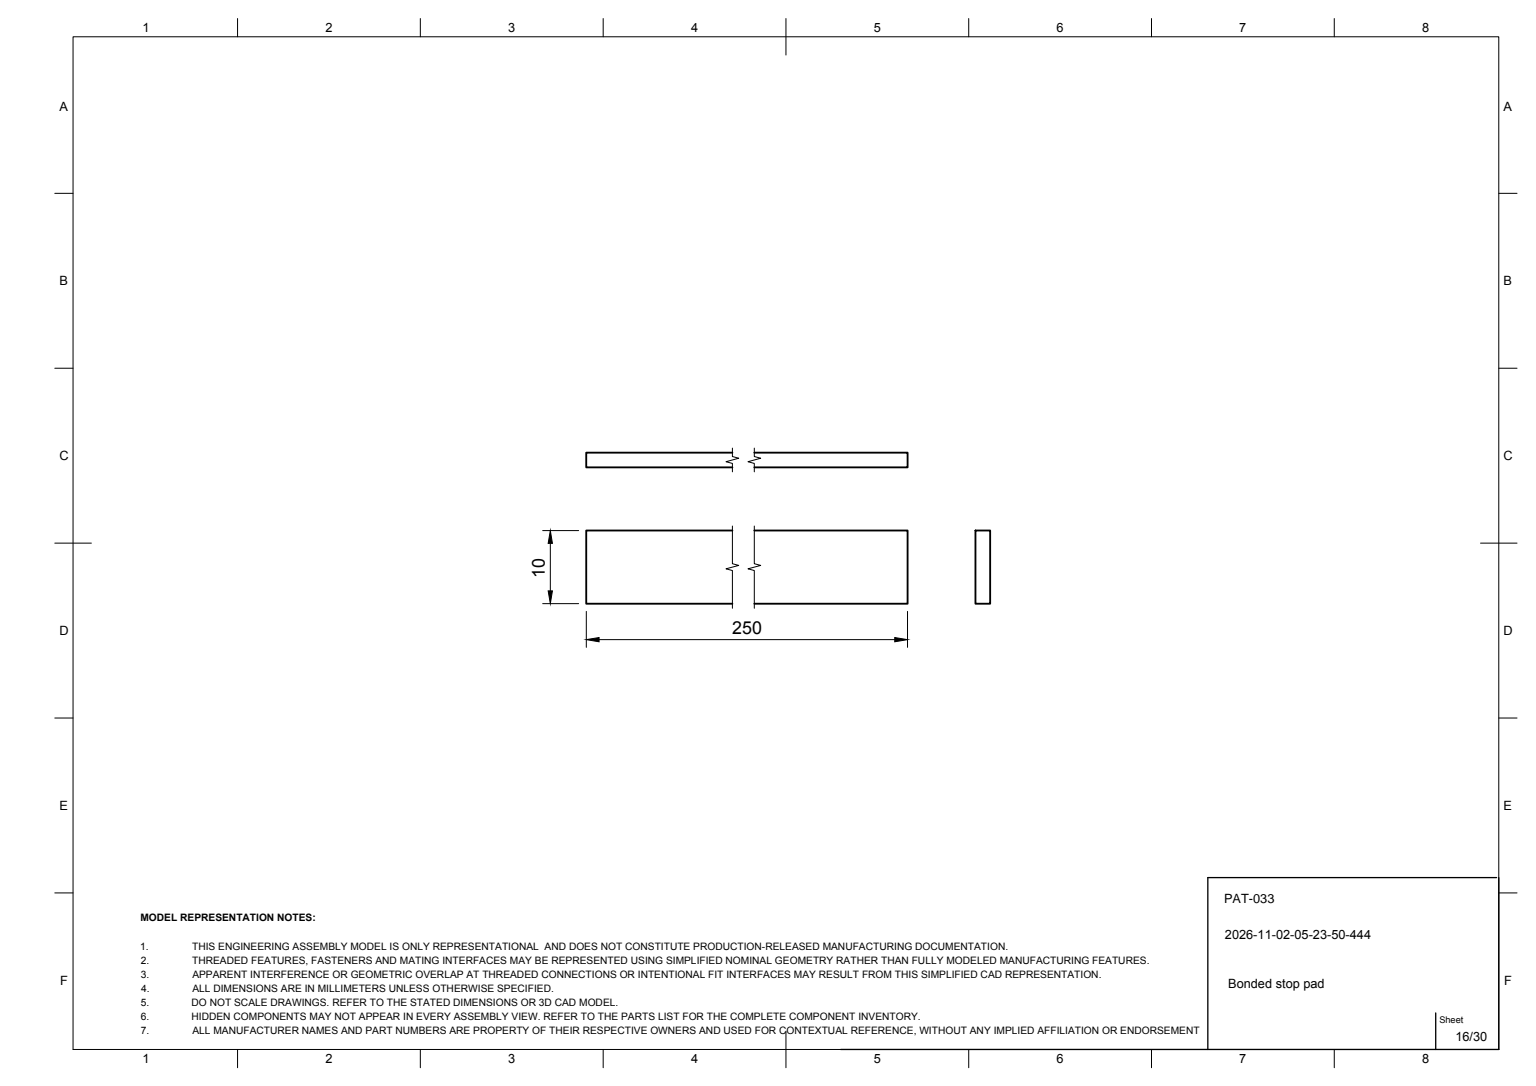
ISO-10303-21;
HEADER;
/* Generated by software containing ST-Developer
 * from STEP Tools, Inc. (www.steptools.com) 
 */

FILE_DESCRIPTION(
/* description */ ('Dual-rail gantry carriage'),
/* implementation_level */ '2;1');

FILE_NAME(
/* name */ 'Bonded stop pad.step',
/* time_stamp */ '2026-10-27T10:49:15-07:00',
/* author */ (''),
/* organization */ (''),
/* preprocessor_version */ 'ST-DEVELOPER v20.2',
/* originating_system */ 'Autodesk Translation Framework v15.17.0.0',
/* authorisation */ '');

FILE_SCHEMA (('AUTOMOTIVE_DESIGN { 1 0 10303 214 3 1 1 }'));
ENDSEC;

DATA;
#10=MECHANICAL_DESIGN_GEOMETRIC_PRESENTATION_REPRESENTATION('',(#596),#12804);
#534=SHAPE_REPRESENTATION_RELATIONSHIP('SRR','None',#13012,#565);
#565=ADVANCED_BREP_SHAPE_REPRESENTATION('',(#627),#12782);
#596=STYLED_ITEM('',(#13261),#627);
#627=MANIFOLD_SOLID_BREP('Body1',#7374);
#834=PLANE('',#7903);
#835=PLANE('',#7904);
#836=PLANE('',#7905);
#837=PLANE('',#7906);
#838=PLANE('',#7907);
#839=PLANE('',#7908);
#1144=FACE_OUTER_BOUND('',#1577,.T.);
#1145=FACE_OUTER_BOUND('',#1578,.T.);
#1146=FACE_OUTER_BOUND('',#1579,.T.);
#1147=FACE_OUTER_BOUND('',#1580,.T.);
#1148=FACE_OUTER_BOUND('',#1581,.T.);
#1149=FACE_OUTER_BOUND('',#1582,.T.);
#1577=EDGE_LOOP('',(#5503,#5504,#5505,#5506));
#1578=EDGE_LOOP('',(#5507,#5508,#5509,#5510));
#1579=EDGE_LOOP('',(#5511,#5512,#5513,#5514));
#1580=EDGE_LOOP('',(#5515,#5516,#5517,#5518));
#1581=EDGE_LOOP('',(#5519,#5520,#5521,#5522));
#1582=EDGE_LOOP('',(#5523,#5524,#5525,#5526));
#2114=LINE('',#11159,#2823);
#2115=LINE('',#11161,#2824);
#2116=LINE('',#11163,#2825);
#2117=LINE('',#11164,#2826);
#2118=LINE('',#11167,#2827);
#2119=LINE('',#11169,#2828);
#2120=LINE('',#11170,#2829);
#2121=LINE('',#11173,#2830);
#2122=LINE('',#11175,#2831);
#2123=LINE('',#11176,#2832);
#2124=LINE('',#11178,#2833);
#2125=LINE('',#11179,#2834);
#2823=VECTOR('',#8979,1.);
#2824=VECTOR('',#8980,1.);
#2825=VECTOR('',#8981,1.);
#2826=VECTOR('',#8982,1.);
#2827=VECTOR('',#8985,1.);
#2828=VECTOR('',#8986,1.);
#2829=VECTOR('',#8987,1.);
#2830=VECTOR('',#8990,1.);
#2831=VECTOR('',#8991,1.);
#2832=VECTOR('',#8992,1.);
#2833=VECTOR('',#8995,1.);
#2834=VECTOR('',#8996,1.);
#3706=VERTEX_POINT('',#11157);
#3707=VERTEX_POINT('',#11158);
#3708=VERTEX_POINT('',#11160);
#3709=VERTEX_POINT('',#11162);
#3710=VERTEX_POINT('',#11166);
#3711=VERTEX_POINT('',#11168);
#3712=VERTEX_POINT('',#11172);
#3713=VERTEX_POINT('',#11174);
#4374=EDGE_CURVE('',#3706,#3707,#2114,.T.);
#4375=EDGE_CURVE('',#3707,#3708,#2115,.T.);
#4376=EDGE_CURVE('',#3709,#3708,#2116,.T.);
#4377=EDGE_CURVE('',#3706,#3709,#2117,.T.);
#4378=EDGE_CURVE('',#3710,#3706,#2118,.T.);
#4379=EDGE_CURVE('',#3711,#3709,#2119,.T.);
#4380=EDGE_CURVE('',#3710,#3711,#2120,.T.);
#4381=EDGE_CURVE('',#3712,#3710,#2121,.T.);
#4382=EDGE_CURVE('',#3713,#3711,#2122,.T.);
#4383=EDGE_CURVE('',#3712,#3713,#2123,.T.);
#4384=EDGE_CURVE('',#3707,#3712,#2124,.T.);
#4385=EDGE_CURVE('',#3708,#3713,#2125,.T.);
#5503=ORIENTED_EDGE('',*,*,#4374,.T.);
#5504=ORIENTED_EDGE('',*,*,#4375,.T.);
#5505=ORIENTED_EDGE('',*,*,#4376,.F.);
#5506=ORIENTED_EDGE('',*,*,#4377,.F.);
#5507=ORIENTED_EDGE('',*,*,#4378,.T.);
#5508=ORIENTED_EDGE('',*,*,#4377,.T.);
#5509=ORIENTED_EDGE('',*,*,#4379,.F.);
#5510=ORIENTED_EDGE('',*,*,#4380,.F.);
#5511=ORIENTED_EDGE('',*,*,#4381,.T.);
#5512=ORIENTED_EDGE('',*,*,#4380,.T.);
#5513=ORIENTED_EDGE('',*,*,#4382,.F.);
#5514=ORIENTED_EDGE('',*,*,#4383,.F.);
#5515=ORIENTED_EDGE('',*,*,#4384,.T.);
#5516=ORIENTED_EDGE('',*,*,#4383,.T.);
#5517=ORIENTED_EDGE('',*,*,#4385,.F.);
#5518=ORIENTED_EDGE('',*,*,#4375,.F.);
#5519=ORIENTED_EDGE('',*,*,#4385,.T.);
#5520=ORIENTED_EDGE('',*,*,#4382,.T.);
#5521=ORIENTED_EDGE('',*,*,#4379,.T.);
#5522=ORIENTED_EDGE('',*,*,#4376,.T.);
#5523=ORIENTED_EDGE('',*,*,#4384,.F.);
#5524=ORIENTED_EDGE('',*,*,#4374,.F.);
#5525=ORIENTED_EDGE('',*,*,#4378,.F.);
#5526=ORIENTED_EDGE('',*,*,#4381,.F.);
#7070=ADVANCED_FACE('',(#1144),#834,.T.);
#7071=ADVANCED_FACE('',(#1145),#835,.T.);
#7072=ADVANCED_FACE('',(#1146),#836,.T.);
#7073=ADVANCED_FACE('',(#1147),#837,.T.);
#7074=ADVANCED_FACE('',(#1148),#838,.T.);
#7075=ADVANCED_FACE('',(#1149),#839,.F.);
#7374=CLOSED_SHELL('',(#7070,#7071,#7072,#7073,#7074,#7075));
#7902=AXIS2_PLACEMENT_3D('',#11155,#8975,#8976);
#7903=AXIS2_PLACEMENT_3D('',#11156,#8977,#8978);
#7904=AXIS2_PLACEMENT_3D('',#11165,#8983,#8984);
#7905=AXIS2_PLACEMENT_3D('',#11171,#8988,#8989);
#7906=AXIS2_PLACEMENT_3D('',#11177,#8993,#8994);
#7907=AXIS2_PLACEMENT_3D('',#11180,#8997,#8998);
#7908=AXIS2_PLACEMENT_3D('',#11181,#8999,#9000);
#8975=DIRECTION('axis',(0.,0.,1.));
#8976=DIRECTION('refdir',(1.,0.,0.));
#8977=DIRECTION('center_axis',(0.,1.,0.));
#8978=DIRECTION('ref_axis',(-1.,0.,0.));
#8979=DIRECTION('',(-1.,0.,0.));
#8980=DIRECTION('',(0.,0.,1.));
#8981=DIRECTION('',(-1.,0.,0.));
#8982=DIRECTION('',(0.,0.,1.));
#8983=DIRECTION('center_axis',(1.,0.,0.));
#8984=DIRECTION('ref_axis',(0.,1.,0.));
#8985=DIRECTION('',(0.,1.,0.));
#8986=DIRECTION('',(0.,1.,0.));
#8987=DIRECTION('',(0.,0.,1.));
#8988=DIRECTION('center_axis',(0.,-1.,0.));
#8989=DIRECTION('ref_axis',(1.,0.,0.));
#8990=DIRECTION('',(1.,0.,0.));
#8991=DIRECTION('',(1.,0.,0.));
#8992=DIRECTION('',(0.,0.,1.));
#8993=DIRECTION('center_axis',(-1.,0.,0.));
#8994=DIRECTION('ref_axis',(0.,-1.,0.));
#8995=DIRECTION('',(0.,-1.,0.));
#8996=DIRECTION('',(0.,-1.,0.));
#8997=DIRECTION('center_axis',(0.,0.,1.));
#8998=DIRECTION('ref_axis',(1.,0.,0.));
#8999=DIRECTION('center_axis',(0.,0.,1.));
#9000=DIRECTION('ref_axis',(1.,0.,0.));
#11155=CARTESIAN_POINT('',(0.,0.,0.));
#11156=CARTESIAN_POINT('Origin',(8.2,12.5,5.2));
#11157=CARTESIAN_POINT('',(8.2,12.5,5.2));
#11158=CARTESIAN_POINT('',(8.,12.5,5.2));
#11159=CARTESIAN_POINT('',(8.2,12.5,5.2));
#11160=CARTESIAN_POINT('',(8.,12.5,6.2));
#11161=CARTESIAN_POINT('',(8.,12.5,5.2));
#11162=CARTESIAN_POINT('',(8.2,12.5,6.2));
#11163=CARTESIAN_POINT('',(8.2,12.5,6.2));
#11164=CARTESIAN_POINT('',(8.2,12.5,5.2));
#11165=CARTESIAN_POINT('Origin',(8.2,-12.5,5.2));
#11166=CARTESIAN_POINT('',(8.2,-12.5,5.2));
#11167=CARTESIAN_POINT('',(8.2,-12.5,5.2));
#11168=CARTESIAN_POINT('',(8.2,-12.5,6.2));
#11169=CARTESIAN_POINT('',(8.2,-12.5,6.2));
#11170=CARTESIAN_POINT('',(8.2,-12.5,5.2));
#11171=CARTESIAN_POINT('Origin',(8.,-12.5,5.2));
#11172=CARTESIAN_POINT('',(8.,-12.5,5.2));
#11173=CARTESIAN_POINT('',(8.,-12.5,5.2));
#11174=CARTESIAN_POINT('',(8.,-12.5,6.2));
#11175=CARTESIAN_POINT('',(8.,-12.5,6.2));
#11176=CARTESIAN_POINT('',(8.,-12.5,5.2));
#11177=CARTESIAN_POINT('Origin',(8.,12.5,5.2));
#11178=CARTESIAN_POINT('',(8.,12.5,5.2));
#11179=CARTESIAN_POINT('',(8.,12.5,6.2));
#11180=CARTESIAN_POINT('Origin',(8.1,0.,6.2));
#11181=CARTESIAN_POINT('Origin',(8.1,0.,5.2));
#12746=UNCERTAINTY_MEASURE_WITH_UNIT(LENGTH_MEASURE(0.001),#12805,
'DISTANCE_ACCURACY_VALUE',
'Maximum model space distance between geometric entities at asserted c
onnectivities');
#12768=UNCERTAINTY_MEASURE_WITH_UNIT(LENGTH_MEASURE(0.001),#12805,
'DISTANCE_ACCURACY_VALUE',
'Maximum model space distance between geometric entities at asserted c
onnectivities');
#12782=(
GEOMETRIC_REPRESENTATION_CONTEXT(3)
GLOBAL_UNCERTAINTY_ASSIGNED_CONTEXT((#12746))
GLOBAL_UNIT_ASSIGNED_CONTEXT((#12805,#12807,#12808))
REPRESENTATION_CONTEXT('','3D')
);
#12804=(
GEOMETRIC_REPRESENTATION_CONTEXT(3)
GLOBAL_UNCERTAINTY_ASSIGNED_CONTEXT((#12768))
GLOBAL_UNIT_ASSIGNED_CONTEXT((#12805,#12807,#12808))
REPRESENTATION_CONTEXT('','3D')
);
#12805=(
LENGTH_UNIT()
NAMED_UNIT(*)
SI_UNIT(.CENTI.,.METRE.)
);
#12807=(
NAMED_UNIT(*)
PLANE_ANGLE_UNIT()
SI_UNIT($,.RADIAN.)
);
#12808=(
NAMED_UNIT(*)
SI_UNIT($,.STERADIAN.)
SOLID_ANGLE_UNIT()
);
#12822=SHAPE_DEFINITION_REPRESENTATION(#12857,#13012);
#12857=PRODUCT_DEFINITION_SHAPE('',$,#13048);
#13012=SHAPE_REPRESENTATION('',(#7902),#12782);
#13034=PRODUCT_DEFINITION_CONTEXT('part definition',#13141,'design');
#13048=PRODUCT_DEFINITION('Bonded stop pad','Bonded stop pad',#13083,#13034);
#13083=PRODUCT_DEFINITION_FORMATION('',$,#13156);
#13141=APPLICATION_CONTEXT(
'Core Data for Automotive Mechanical Design Process');
#13142=PRODUCT_CONTEXT('part definition',#13141,'mechanical');
#13156=PRODUCT('Bonded stop pad','Bonded stop pad','Bonded stop pad',(#13142));
#13255=COLOUR_RGB('Off White',0.89,0.88,0.83);
#13256=FILL_AREA_STYLE_COLOUR('',#13255);
#13257=FILL_AREA_STYLE('',(#13256));
#13258=SURFACE_STYLE_FILL_AREA(#13257);
#13259=SURFACE_SIDE_STYLE('',(#13258));
#13260=SURFACE_STYLE_USAGE(.BOTH.,#13259);
#13261=PRESENTATION_STYLE_ASSIGNMENT((#13260));
ENDSEC;
END-ISO-10303-21;
